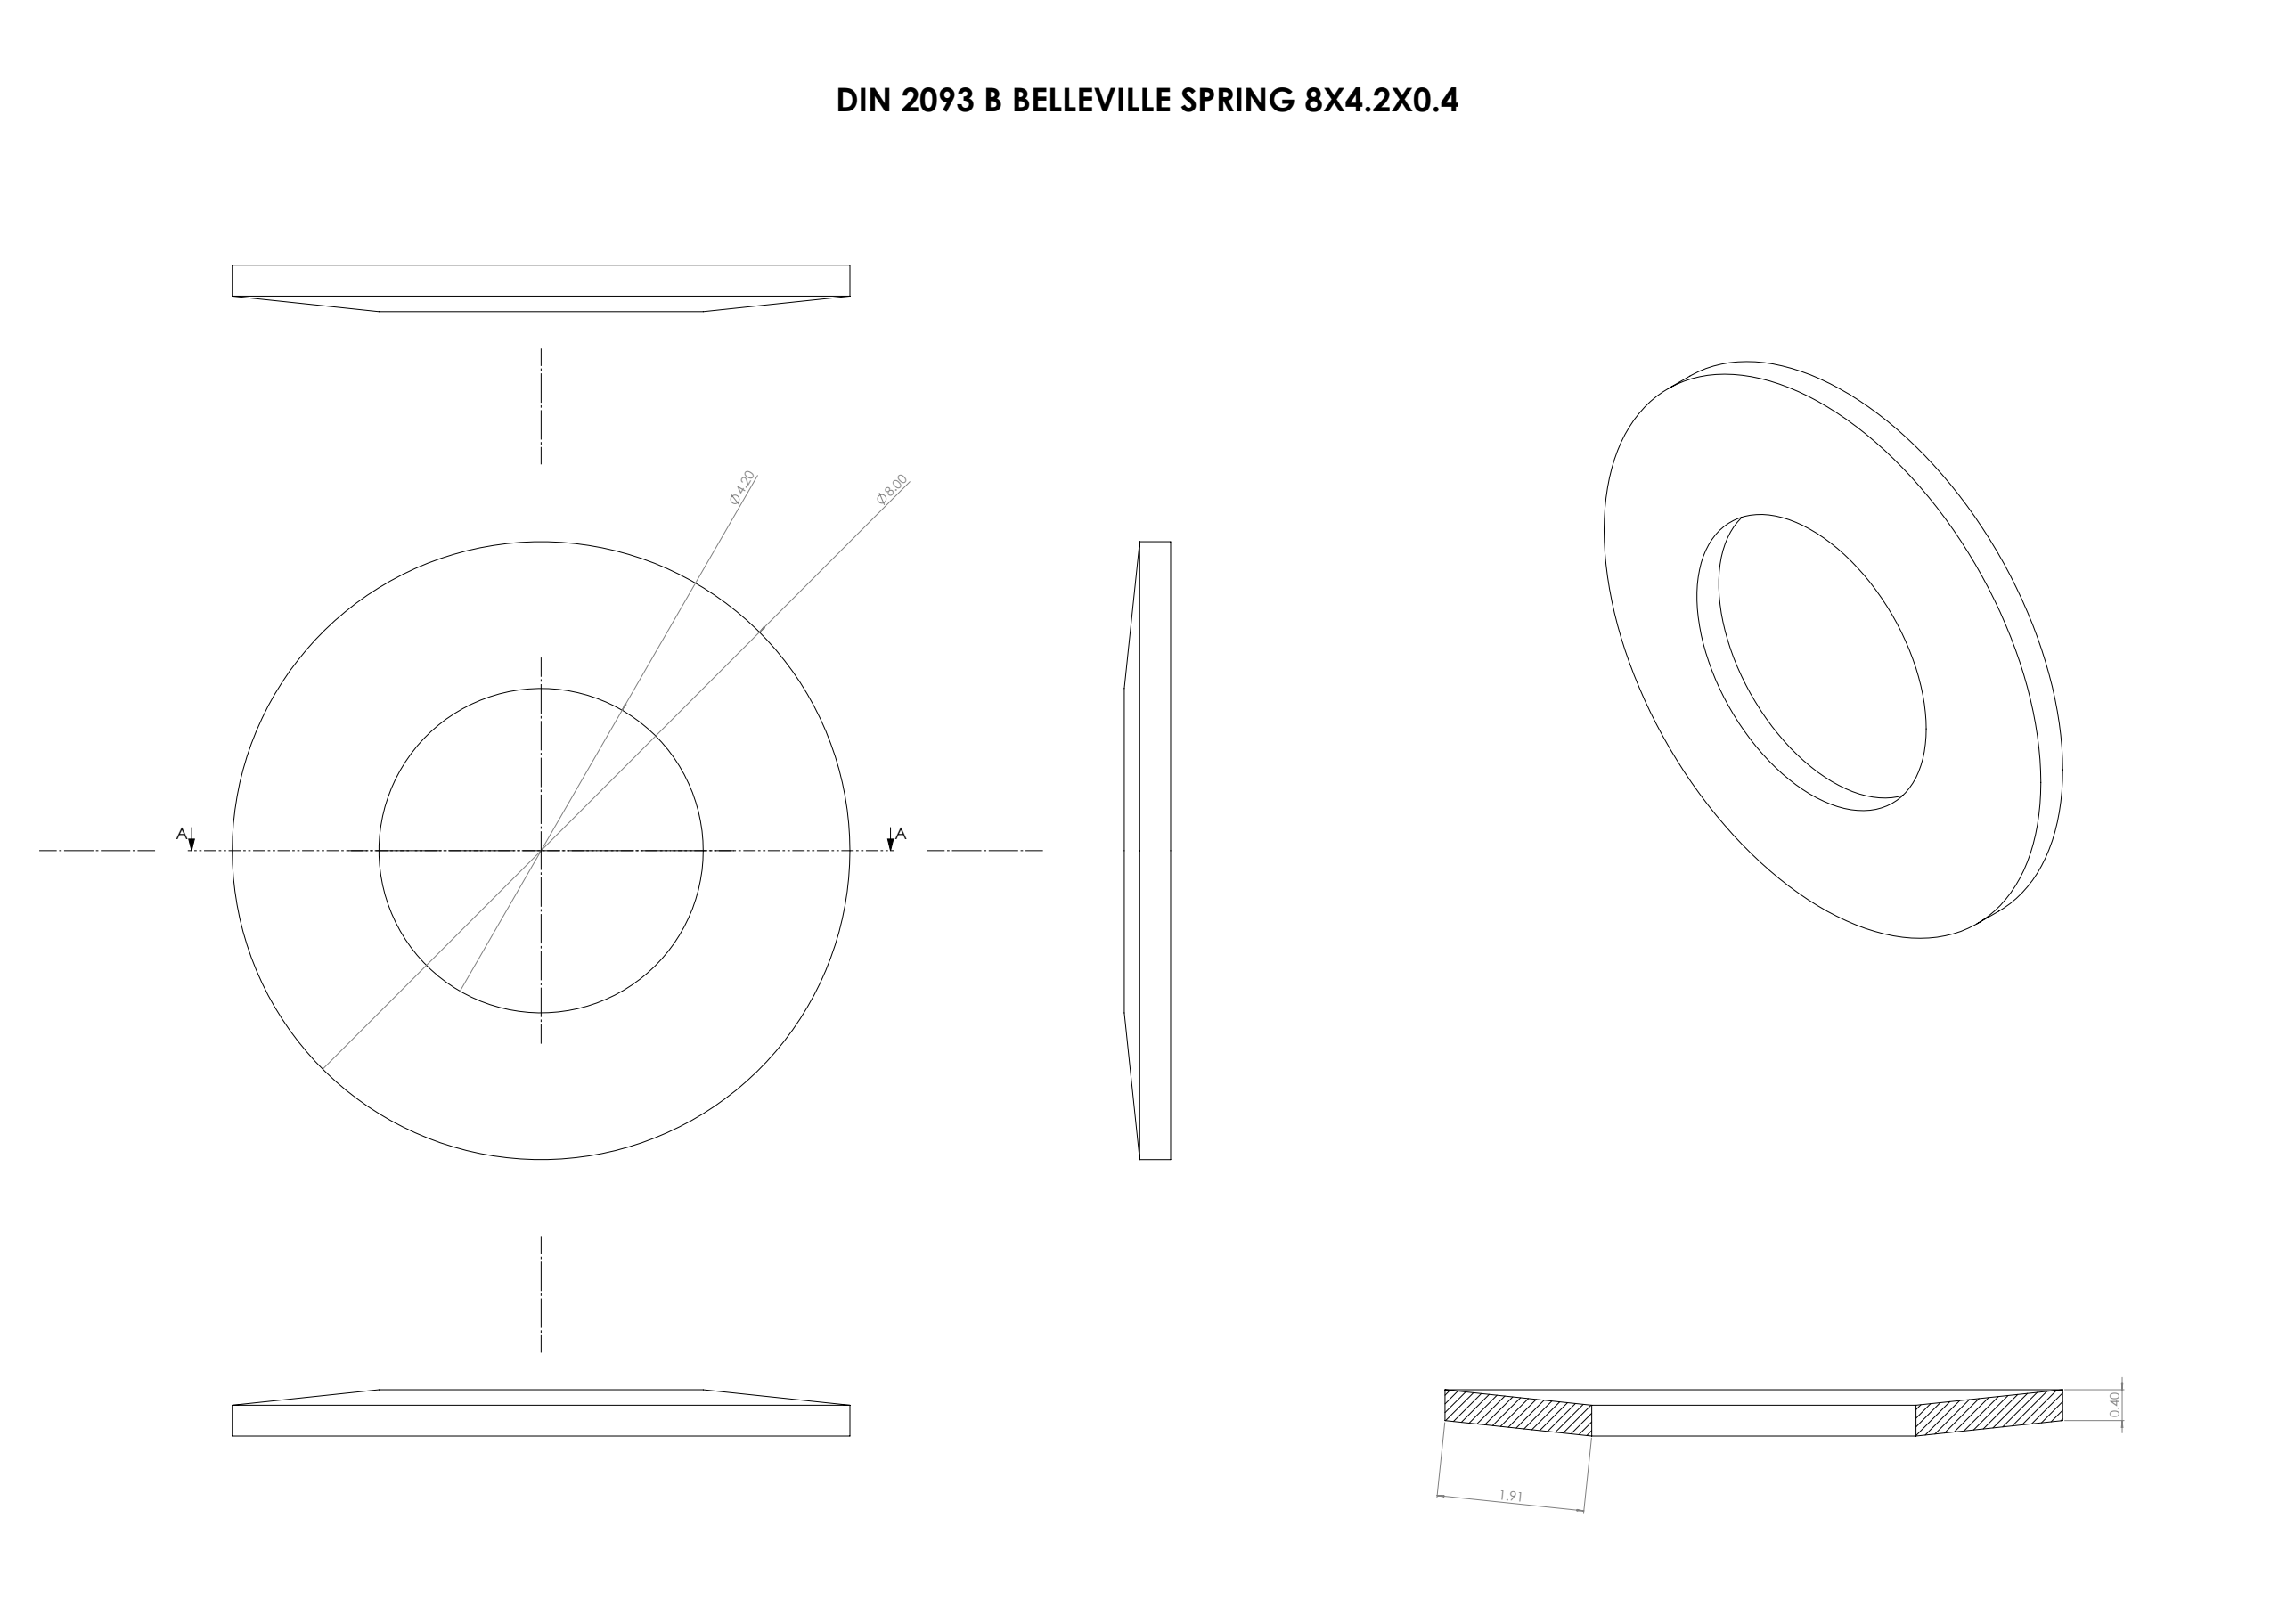
ISO-10303-21;
HEADER;
/* Generated by software containing ST-Developer
 * from STEP Tools, Inc. (www.steptools.com) 
 */

FILE_DESCRIPTION(
/* description */ (''),
/* implementation_level */ '2;1');

FILE_NAME(
/* name */ '10_DIN_2093_B_Belleville_Spring_8x4.2x0.4.step',
/* time_stamp */ '2026-10-19T22:59:19-07:00',
/* author */ (''),
/* organization */ (''),
/* preprocessor_version */ 'ST-DEVELOPER v20.2',
/* originating_system */ 'Autodesk Translation Framework v15.15.0.0',
/* authorisation */ '');

FILE_SCHEMA (('AUTOMOTIVE_DESIGN { 1 0 10303 214 3 1 1 }'));
ENDSEC;

DATA;
#10=MECHANICAL_DESIGN_GEOMETRIC_PRESENTATION_REPRESENTATION('',(#922),#53650);
#890=SHAPE_REPRESENTATION_RELATIONSHIP('SRR','None',#53735,#906);
#906=ADVANCED_BREP_SHAPE_REPRESENTATION('',(#938),#53645);
#922=STYLED_ITEM('',(#53958),#938);
#938=MANIFOLD_SOLID_BREP('Disc Spring',#23314);
#1051=CYLINDRICAL_SURFACE('',#24587,0.21);
#1052=CYLINDRICAL_SURFACE('',#24592,0.4);
#2852=FACE_OUTER_BOUND('',#4317,.T.);
#2853=FACE_OUTER_BOUND('',#4318,.T.);
#2854=FACE_OUTER_BOUND('',#4319,.T.);
#2855=FACE_OUTER_BOUND('',#4320,.T.);
#4317=EDGE_LOOP('',(#17781,#17782,#17783,#17784));
#4318=EDGE_LOOP('',(#17785,#17786,#17787,#17788));
#4319=EDGE_LOOP('',(#17789,#17790,#17791,#17792));
#4320=EDGE_LOOP('',(#17793,#17794,#17795,#17796));
#5527=CIRCLE('',#24588,0.21);
#5528=CIRCLE('',#24589,0.21);
#5529=CIRCLE('',#24591,0.4);
#5530=CIRCLE('',#24593,0.4);
#6694=LINE('',#36144,#8539);
#6695=LINE('',#36148,#8540);
#6696=LINE('',#36153,#8541);
#6697=LINE('',#36155,#8542);
#8539=VECTOR('',#28682,0.21);
#8540=VECTOR('',#28687,0.305);
#8541=VECTOR('',#28694,0.4);
#8542=VECTOR('',#28697,0.305);
#10382=VERTEX_POINT('',#36141);
#10383=VERTEX_POINT('',#36143);
#10384=VERTEX_POINT('',#36147);
#10385=VERTEX_POINT('',#36151);
#13068=EDGE_CURVE('',#10382,#10382,#5527,.T.);
#13069=EDGE_CURVE('',#10382,#10383,#6694,.T.);
#13070=EDGE_CURVE('',#10383,#10383,#5528,.T.);
#13071=EDGE_CURVE('',#10383,#10384,#6695,.T.);
#13072=EDGE_CURVE('',#10384,#10384,#5529,.T.);
#13073=EDGE_CURVE('',#10385,#10385,#5530,.T.);
#13074=EDGE_CURVE('',#10385,#10384,#6696,.T.);
#13075=EDGE_CURVE('',#10382,#10385,#6697,.T.);
#17781=ORIENTED_EDGE('',*,*,#13068,.T.);
#17782=ORIENTED_EDGE('',*,*,#13069,.T.);
#17783=ORIENTED_EDGE('',*,*,#13070,.F.);
#17784=ORIENTED_EDGE('',*,*,#13069,.F.);
#17785=ORIENTED_EDGE('',*,*,#13070,.T.);
#17786=ORIENTED_EDGE('',*,*,#13071,.T.);
#17787=ORIENTED_EDGE('',*,*,#13072,.F.);
#17788=ORIENTED_EDGE('',*,*,#13071,.F.);
#17789=ORIENTED_EDGE('',*,*,#13073,.F.);
#17790=ORIENTED_EDGE('',*,*,#13074,.T.);
#17791=ORIENTED_EDGE('',*,*,#13072,.T.);
#17792=ORIENTED_EDGE('',*,*,#13074,.F.);
#17793=ORIENTED_EDGE('',*,*,#13068,.F.);
#17794=ORIENTED_EDGE('',*,*,#13075,.T.);
#17795=ORIENTED_EDGE('',*,*,#13073,.T.);
#17796=ORIENTED_EDGE('',*,*,#13075,.F.);
#21957=CONICAL_SURFACE('',#24590,0.305,1.46591938806466);
#21958=CONICAL_SURFACE('',#24594,0.305,1.46591938806466);
#22591=ADVANCED_FACE('',(#2852),#1051,.F.);
#22592=ADVANCED_FACE('',(#2853),#21957,.F.);
#22593=ADVANCED_FACE('',(#2854),#1052,.T.);
#22594=ADVANCED_FACE('',(#2855),#21958,.T.);
#23314=CLOSED_SHELL('',(#22591,#22592,#22593,#22594));
#24586=AXIS2_PLACEMENT_3D('',#36139,#28676,#28677);
#24587=AXIS2_PLACEMENT_3D('',#36140,#28678,#28679);
#24588=AXIS2_PLACEMENT_3D('',#36142,#28680,#28681);
#24589=AXIS2_PLACEMENT_3D('',#36145,#28683,#28684);
#24590=AXIS2_PLACEMENT_3D('',#36146,#28685,#28686);
#24591=AXIS2_PLACEMENT_3D('',#36149,#28688,#28689);
#24592=AXIS2_PLACEMENT_3D('',#36150,#28690,#28691);
#24593=AXIS2_PLACEMENT_3D('',#36152,#28692,#28693);
#24594=AXIS2_PLACEMENT_3D('',#36154,#28695,#28696);
#28676=DIRECTION('axis',(0.,0.,1.));
#28677=DIRECTION('refdir',(1.,0.,0.));
#28678=DIRECTION('center_axis',(0.,0.,1.));
#28679=DIRECTION('ref_axis',(1.,0.,0.));
#28680=DIRECTION('center_axis',(0.,0.,1.));
#28681=DIRECTION('ref_axis',(1.,0.,0.));
#28682=DIRECTION('',(0.,0.,-1.));
#28683=DIRECTION('center_axis',(0.,0.,1.));
#28684=DIRECTION('ref_axis',(1.,0.,0.));
#28685=DIRECTION('center_axis',(0.,0.,-1.));
#28686=DIRECTION('ref_axis',(1.,0.,0.));
#28687=DIRECTION('',(-0.994505452921406,-1.21791791965479E-16,-0.104684784518043));
#28688=DIRECTION('center_axis',(0.,0.,1.));
#28689=DIRECTION('ref_axis',(1.,0.,0.));
#28690=DIRECTION('center_axis',(0.,0.,1.));
#28691=DIRECTION('ref_axis',(1.,0.,0.));
#28692=DIRECTION('center_axis',(0.,0.,1.));
#28693=DIRECTION('ref_axis',(1.,0.,0.));
#28694=DIRECTION('',(0.,0.,-1.));
#28695=DIRECTION('center_axis',(0.,0.,-1.));
#28696=DIRECTION('ref_axis',(1.,0.,0.));
#28697=DIRECTION('',(-0.994505452921406,-1.21791791965479E-16,-0.104684784518043));
#36139=CARTESIAN_POINT('',(0.,0.,0.));
#36140=CARTESIAN_POINT('Origin',(0.,0.,0.04));
#36141=CARTESIAN_POINT('',(-0.21,-2.57175827820944E-17,0.06));
#36142=CARTESIAN_POINT('Origin',(0.,0.,0.06));
#36143=CARTESIAN_POINT('',(-0.21,-2.57175827820944E-17,0.02));
#36144=CARTESIAN_POINT('',(-0.21,-2.57175827820944E-17,0.04));
#36145=CARTESIAN_POINT('Origin',(0.,0.,0.02));
#36146=CARTESIAN_POINT('Origin',(0.,0.,0.01));
#36147=CARTESIAN_POINT('',(-0.4,-4.89858719658941E-17,3.46944695195361E-18));
#36148=CARTESIAN_POINT('',(-0.305,-3.73517273739943E-17,0.01));
#36149=CARTESIAN_POINT('Origin',(0.,0.,0.));
#36150=CARTESIAN_POINT('Origin',(0.,0.,0.02));
#36151=CARTESIAN_POINT('',(-0.4,-4.89858719658941E-17,0.04));
#36152=CARTESIAN_POINT('Origin',(0.,0.,0.04));
#36153=CARTESIAN_POINT('',(-0.4,-4.89858719658941E-17,0.02));
#36154=CARTESIAN_POINT('Origin',(0.,0.,0.05));
#36155=CARTESIAN_POINT('',(-0.305,-3.73517273739943E-17,0.05));
#53627=UNCERTAINTY_MEASURE_WITH_UNIT(LENGTH_MEASURE(0.001),#53651,
'DISTANCE_ACCURACY_VALUE',
'Maximum model space distance between geometric entities at asserted c
onnectivities');
#53632=UNCERTAINTY_MEASURE_WITH_UNIT(LENGTH_MEASURE(0.001),#53651,
'DISTANCE_ACCURACY_VALUE',
'Maximum model space distance between geometric entities at asserted c
onnectivities');
#53645=(
GEOMETRIC_REPRESENTATION_CONTEXT(3)
GLOBAL_UNCERTAINTY_ASSIGNED_CONTEXT((#53627))
GLOBAL_UNIT_ASSIGNED_CONTEXT((#53651,#53653,#53654))
REPRESENTATION_CONTEXT('','3D')
);
#53650=(
GEOMETRIC_REPRESENTATION_CONTEXT(3)
GLOBAL_UNCERTAINTY_ASSIGNED_CONTEXT((#53632))
GLOBAL_UNIT_ASSIGNED_CONTEXT((#53651,#53653,#53654))
REPRESENTATION_CONTEXT('','3D')
);
#53651=(
LENGTH_UNIT()
NAMED_UNIT(*)
SI_UNIT(.CENTI.,.METRE.)
);
#53653=(
NAMED_UNIT(*)
PLANE_ANGLE_UNIT()
SI_UNIT($,.RADIAN.)
);
#53654=(
NAMED_UNIT(*)
SI_UNIT($,.STERADIAN.)
SOLID_ANGLE_UNIT()
);
#53667=SHAPE_DEFINITION_REPRESENTATION(#53684,#53735);
#53684=PRODUCT_DEFINITION_SHAPE('',$,#53753);
#53735=SHAPE_REPRESENTATION('',(#24586),#53645);
#53740=PRODUCT_DEFINITION_CONTEXT('part definition',#53793,'design');
#53753=PRODUCT_DEFINITION('2026-10-18-22-44-45-955',
'10_DIN_2093_B_Belleville_Spring_8x4.2x0.4',#53770,#53740);
#53770=PRODUCT_DEFINITION_FORMATION('',$,#53807);
#53793=APPLICATION_CONTEXT(
'Core Data for Automotive Mechanical Design Process');
#53794=PRODUCT_CONTEXT('part definition',#53793,'mechanical');
#53807=PRODUCT('2026-10-18-22-44-45-955',
'10_DIN_2093_B_Belleville_Spring_8x4.2x0.4',$,(#53794));
#53952=COLOUR_RGB('Grey',0.48,0.52,0.57);
#53953=FILL_AREA_STYLE_COLOUR('',#53952);
#53954=FILL_AREA_STYLE('',(#53953));
#53955=SURFACE_STYLE_FILL_AREA(#53954);
#53956=SURFACE_SIDE_STYLE('',(#53955));
#53957=SURFACE_STYLE_USAGE(.BOTH.,#53956);
#53958=PRESENTATION_STYLE_ASSIGNMENT((#53957));
ENDSEC;
END-ISO-10303-21;
